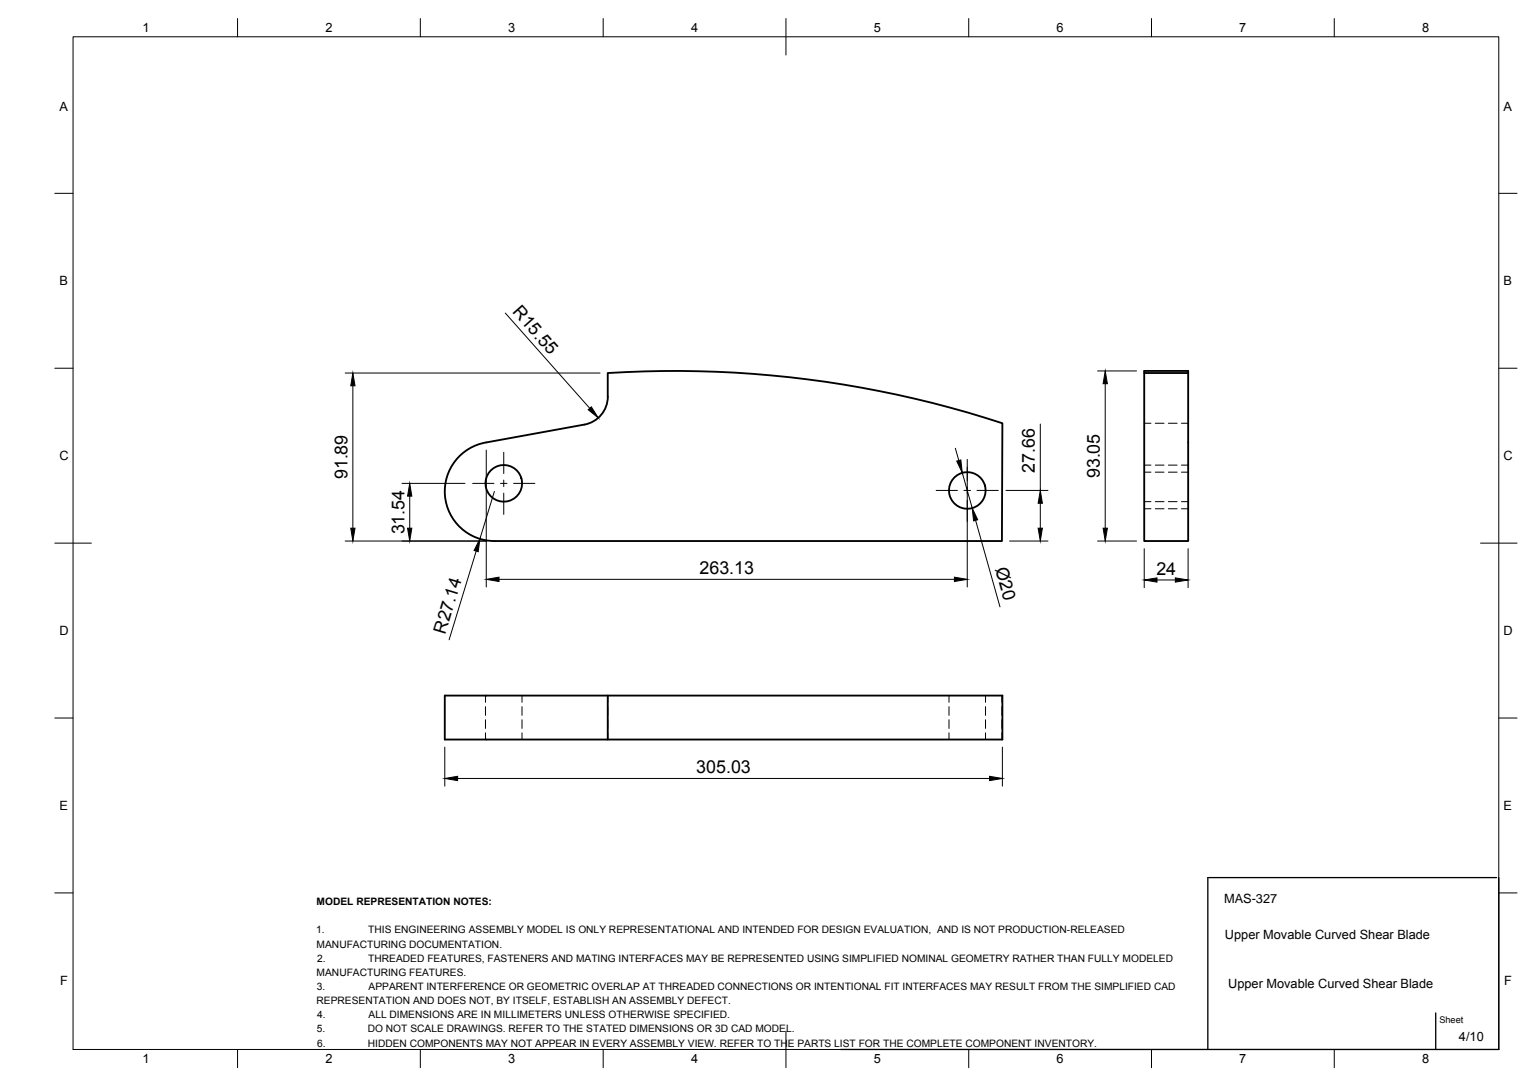
ISO-10303-21;
HEADER;
FILE_DESCRIPTION (('STEP AP214'),
    '1' );
FILE_NAME ('Upper Movable Curved Shear Blade.step',
    '2026-10-06T22:16:42',
    ( '' ),
    ( '' ),
    'SwSTEP 2.0',
    'SolidWorks 2025',
    '' );
FILE_SCHEMA (( 'AUTOMOTIVE_DESIGN' ));
ENDSEC;

DATA;
#48=FACE_BOUND ( 'NONE', #8175, .T. ) ;
#84=VECTOR ( 'NONE', #11009, 1000.000000000000000 ) ;
#209=CIRCLE ( 'NONE', #14661, 576.1986910693910886 ) ;
#225=ORIENTED_EDGE ( 'NONE', *, *, #21350, .F. ) ;
#238=EDGE_CURVE ( 'NONE', #951, #16393, #2471, .T. ) ;
#293=DIRECTION ( 'NONE',  ( -0.9609212714474144601, -0.2768218020313507610, 0.000000000000000000 ) ) ;
#337=ORIENTED_EDGE ( 'NONE', *, *, #13071, .F. ) ;
#354=DIRECTION ( 'NONE',  ( 0.000000000000000000, 0.000000000000000000, 1.000000000000000000 ) ) ;
#375=CLOSED_SHELL ( 'NONE', ( #8062, #8739, #16372, #2106, #6229, #2878, #10037, #18884, #18118, #3960, #13156, #6514, #20224, #19647 ) ) ;
#400=DIRECTION ( 'NONE',  ( 1.000000000000000000, 0.000000000000000000, 0.000000000000000000 ) ) ;
#488=VERTEX_POINT ( 'NONE', #17503 ) ;
#507=CARTESIAN_POINT ( 'NONE',  ( 180.1254907973641934, 54.87273858953557237, 4.000000000000021316 ) ) ;
#570=ORIENTED_EDGE ( 'NONE', *, *, #6351, .T. ) ;
#625=EDGE_LOOP ( 'NONE', ( #14044, #7065, #9180, #16970 ) ) ;
#792=EDGE_LOOP ( 'NONE', ( #7745, #13828, #225, #21173 ) ) ;
#896=ORIENTED_EDGE ( 'NONE', *, *, #16906, .F. ) ;
#935=DIRECTION ( 'NONE',  ( 1.000000000000000000, 0.000000000000000000, 0.000000000000000000 ) ) ;
#951=VERTEX_POINT ( 'NONE', #1744 ) ;
#964=CYLINDRICAL_SURFACE ( 'NONE', #11411, 10.00000000000000888 ) ;
#975=AXIS2_PLACEMENT_3D ( 'NONE', #5264, #5469, #6716 ) ;
#1029=FACE_OUTER_BOUND ( 'NONE', #6208, .T. ) ;
#1042=STYLED_ITEM ( 'NONE', ( #2053 ), #21529 ) ;
#1044=CARTESIAN_POINT ( 'NONE',  ( 161.4773229304660731, 84.89323405393692212, 4.000000000000021316 ) ) ;
#1179=DIRECTION ( 'NONE',  ( -0.000000000000000000, -0.000000000000000000, -1.000000000000000000 ) ) ;
#1205=FACE_OUTER_BOUND ( 'NONE', #8630, .T. ) ;
#1253=DIRECTION ( 'NONE',  ( -0.9599098561846887145, -0.2803088796301151375, 0.000000000000000000 ) ) ;
#1266=AXIS2_PLACEMENT_3D ( 'NONE', #2104, #12019, #2214 ) ;
#1272=EDGE_CURVE ( 'NONE', #951, #12140, #21577, .T. ) ;
#1305=VERTEX_POINT ( 'NONE', #9789 ) ;
#1307=FACE_OUTER_BOUND ( 'NONE', #18026, .T. ) ;
#1322=VECTOR ( 'NONE', #10602, 1000.000000000000000 ) ;
#1342=AXIS2_PLACEMENT_3D ( 'NONE', #8297, #20202, #15234 ) ;
#1409=APPLICATION_CONTEXT ( 'automotive_design' ) ;
#1477=CARTESIAN_POINT ( 'NONE',  ( 180.1254907973641934, 54.87273858953557237, 4.000000000000021316 ) ) ;
#1578=ORIENTED_EDGE ( 'NONE', *, *, #8963, .T. ) ;
#1633=CIRCLE ( 'NONE', #16042, 9.999999999999994671 ) ;
#1716=ORIENTED_EDGE ( 'NONE', *, *, #20163, .F. ) ;
#1717=EDGE_CURVE ( 'NONE', #16694, #21813, #4400, .T. ) ;
#1744=CARTESIAN_POINT ( 'NONE',  ( -104.7439762501682736, 39.86119447055682485, 4.000000000000021316 ) ) ;
#1816=UNCERTAINTY_MEASURE_WITH_UNIT (LENGTH_MEASURE( 1.000000000000000082E-05 ), #4027, 'distance_accuracy_value', 'NONE');
#1879=ORIENTED_EDGE ( 'NONE', *, *, #19571, .F. ) ;
#1905=VERTEX_POINT ( 'NONE', #7889 ) ;
#1914=EDGE_CURVE ( 'NONE', #10160, #15098, #7604, .T. ) ;
#1954=CARTESIAN_POINT ( 'NONE',  ( -94.10404323627655288, -13.18023274290474767, 4.000000000000021316 ) ) ;
#1980=CARTESIAN_POINT ( 'NONE',  ( 161.4773229304660731, 84.89323405393692212, -19.99999999999997868 ) ) ;
#2053=PRESENTATION_STYLE_ASSIGNMENT (( #7561 ) ) ;
#2104=CARTESIAN_POINT ( 'NONE',  ( -38.21168032741934439, -23.19216891395253910, -19.99999999999997868 ) ) ;
#2106=ADVANCED_FACE ( 'NONE', ( #48, #13498, #17116 ), #16685, .T. ) ;
#2150=ORIENTED_EDGE ( 'NONE', *, *, #9010, .T. ) ;
#2168=CARTESIAN_POINT ( 'NONE',  ( 180.1254907973641934, 54.87273858953557237, 4.000000000000021316 ) ) ;
#2187=VECTOR ( 'NONE', #12158, 1000.000000000000000 ) ;
#2214=DIRECTION ( 'NONE',  ( -1.000000000000000000, 0.000000000000000000, 0.000000000000000000 ) ) ;
#2361=VERTEX_POINT ( 'NONE', #6415 ) ;
#2403=CARTESIAN_POINT ( 'NONE',  ( 0.000000000000000000, 0.000000000000000000, 0.000000000000000000 ) ) ;
#2471=CIRCLE ( 'NONE', #12318, 27.14138364107347812 ) ;
#2487=CYLINDRICAL_SURFACE ( 'NONE', #17723, 10.00000000000000888 ) ;
#2538=CARTESIAN_POINT ( 'NONE',  ( 162.0641828542163125, 116.7231784796025948, -19.99999999999997868 ) ) ;
#2579=DIRECTION ( 'NONE',  ( 0.2768218020313508165, -0.9609212714474144601, 0.000000000000000000 ) ) ;
#2664=EDGE_CURVE ( 'NONE', #10827, #15137, #5819, .T. ) ;
#2733=DIRECTION ( 'NONE',  ( 0.9949940778855791423, 0.09993390301907582873, 0.000000000000000000 ) ) ;
#2843=LINE ( 'NONE', #18047, #84 ) ;
#2876=CIRCLE ( 'NONE', #14842, 9.999999999999994671 ) ;
#2878=ADVANCED_FACE ( 'NONE', ( #1205 ), #16736, .T. ) ;
#3049=DIRECTION ( 'NONE',  ( 1.000000000000000000, 0.000000000000000000, -0.000000000000000000 ) ) ;
#3238=AXIS2_PLACEMENT_3D ( 'NONE', #19808, #9892, #3049 ) ;
#3242=CARTESIAN_POINT ( 'NONE',  ( -101.1064508287285832, 10.96617311717548660, 4.000000000000021316 ) ) ;
#3459=EDGE_LOOP ( 'NONE', ( #7718, #4157, #7317, #15466 ) ) ;
#3466=EDGE_CURVE ( 'NONE', #9506, #10827, #4066, .T. ) ;
#3570=VERTEX_POINT ( 'NONE', #12547 ) ;
#3591=EDGE_CURVE ( 'NONE', #4466, #7553, #14300, .T. ) ;
#3672=ORIENTED_EDGE ( 'NONE', *, *, #238, .T. ) ;
#3713=AXIS2_PLACEMENT_3D ( 'NONE', #9112, #4032, #935 ) ;
#3776=EDGE_LOOP ( 'NONE', ( #15667, #19204 ) ) ;
#3783=ORIENTED_EDGE ( 'NONE', *, *, #14965, .F. ) ;
#3812=ORIENTED_EDGE ( 'NONE', *, *, #238, .F. ) ;
#3867=( GEOMETRIC_REPRESENTATION_CONTEXT ( 3 ) GLOBAL_UNCERTAINTY_ASSIGNED_CONTEXT ( ( #1816 ) ) GLOBAL_UNIT_ASSIGNED_CONTEXT ( ( #4027, #8894, #9109 ) ) REPRESENTATION_CONTEXT ( 'NONE', 'WORKASPACE' ) );
#3877=LINE ( 'NONE', #5737, #1322 ) ;
#3886=PRODUCT_DEFINITION_FORMATION_WITH_SPECIFIED_SOURCE ( 'ANY', '', #9956, .NOT_KNOWN. ) ;
#3924=CARTESIAN_POINT ( 'NONE',  ( 151.4773229304660731, 84.89323405393692212, -19.99999999999997868 ) ) ;
#3942=ORIENTED_EDGE ( 'NONE', *, *, #8167, .F. ) ;
#3960=ADVANCED_FACE ( 'NONE', ( #13848 ), #20583, .T. ) ;
#4027=( LENGTH_UNIT ( ) NAMED_UNIT ( * ) SI_UNIT ( .MILLI., .METRE. ) );
#4029=EDGE_CURVE ( 'NONE', #20969, #10160, #18710, .T. ) ;
#4032=DIRECTION ( 'NONE',  ( 0.000000000000000000, 0.000000000000000000, 1.000000000000000000 ) ) ;
#4041=FACE_OUTER_BOUND ( 'NONE', #14824, .T. ) ;
#4059=DIRECTION ( 'NONE',  ( -0.9949940778855791423, -0.09993390301907582873, 0.000000000000000000 ) ) ;
#4066=LINE ( 'NONE', #21045, #18173 ) ;
#4099=AXIS2_PLACEMENT_3D ( 'NONE', #10030, #8156, #14861 ) ;
#4128=ORIENTED_EDGE ( 'NONE', *, *, #10231, .T. ) ;
#4157=ORIENTED_EDGE ( 'NONE', *, *, #6919, .F. ) ;
#4183=VERTEX_POINT ( 'NONE', #2168 ) ;
#4196=CARTESIAN_POINT ( 'NONE',  ( 151.4773229304660731, 84.89323405393692212, 4.000000000000021316 ) ) ;
#4226=CYLINDRICAL_SURFACE ( 'NONE', #7967, 9.999999999999994671 ) ;
#4231=EDGE_CURVE ( 'NONE', #10160, #10827, #7575, .T. ) ;
#4258=EDGE_CURVE ( 'NONE', #15220, #21430, #19462, .T. ) ;
#4284=PRODUCT_DEFINITION_SHAPE ( 'NONE', 'NONE',  #20915 ) ;
#4327=DIRECTION ( 'NONE',  ( -0.000000000000000000, -0.000000000000000000, -1.000000000000000000 ) ) ;
#4350=CARTESIAN_POINT ( 'NONE',  ( 180.1254907973641934, 54.87273858953557237, -19.99999999999997868 ) ) ;
#4383=ORIENTED_EDGE ( 'NONE', *, *, #6351, .F. ) ;
#4400=CIRCLE ( 'NONE', #3713, 9.999999999999994671 ) ;
#4403=ORIENTED_EDGE ( 'NONE', *, *, #8525, .T. ) ;
#4466=VERTEX_POINT ( 'NONE', #11295 ) ;
#4508=DIRECTION ( 'NONE',  ( -1.000000000000000000, 0.000000000000000000, 0.000000000000000000 ) ) ;
#4562=DIRECTION ( 'NONE',  ( -0.000000000000000000, -0.000000000000000000, -1.000000000000000000 ) ) ;
#4585=FACE_BOUND ( 'NONE', #17508, .T. ) ;
#4591=DIRECTION ( 'NONE',  ( -1.000000000000000000, 0.000000000000000000, 0.000000000000000000 ) ) ;
#4638=AXIS2_PLACEMENT_3D ( 'NONE', #18358, #13178, #19910 ) ;
#4642=DIRECTION ( 'NONE',  ( 1.000000000000000000, 0.000000000000000000, 0.000000000000000000 ) ) ;
#4701=DIRECTION ( 'NONE',  ( -0.000000000000000000, -0.000000000000000000, -1.000000000000000000 ) ) ;
#4739=DIRECTION ( 'NONE',  ( 1.000000000000000000, 0.000000000000000000, 0.000000000000000000 ) ) ;
#4768=DIRECTION ( 'NONE',  ( 0.000000000000000000, 0.000000000000000000, 1.000000000000000000 ) ) ;
#4782=DIRECTION ( 'NONE',  ( 0.000000000000000000, 0.000000000000000000, 1.000000000000000000 ) ) ;
#4806=DIRECTION ( 'NONE',  ( 1.000000000000000000, 0.000000000000000000, 0.000000000000000000 ) ) ;
#4831=CYLINDRICAL_SURFACE ( 'NONE', #9491, 9.999999999999994671 ) ;
#4872=LINE ( 'NONE', #16542, #5060 ) ;
#5060=VECTOR ( 'NONE', #21745, 1000.000000000000000 ) ;
#5264=CARTESIAN_POINT ( 'NONE',  ( -143.7724355939531904, 531.4176628826018032, 4.000000000000021316 ) ) ;
#5334=CARTESIAN_POINT ( 'NONE',  ( -97.23064952102208736, 13.78046159333444720, 4.000000000000021316 ) ) ;
#5357=CARTESIAN_POINT ( 'NONE',  ( -19.70755683829218796, -31.26594044116892590, -19.99999999999997868 ) ) ;
#5385=CARTESIAN_POINT ( 'NONE',  ( -81.10645082872859746, 10.96617311717548837, -19.99999999999997868 ) ) ;
#5436=CARTESIAN_POINT ( 'NONE',  ( -23.27144139456156324, -18.88988604584387332, -19.99999999999997868 ) ) ;
#5462=VECTOR ( 'NONE', #1179, 1000.000000000000000 ) ;
#5469=DIRECTION ( 'NONE',  ( -0.000000000000000000, -0.000000000000000000, -1.000000000000000000 ) ) ;
#5555=EDGE_CURVE ( 'NONE', #13376, #488, #6969, .T. ) ;
#5607=EDGE_CURVE ( 'NONE', #1905, #21813, #3877, .T. ) ;
#5629=VERTEX_POINT ( 'NONE', #2538 ) ;
#5697=ORIENTED_EDGE ( 'NONE', *, *, #11604, .T. ) ;
#5737=CARTESIAN_POINT ( 'NONE',  ( -81.10645082872859746, 10.96617311717548837, 4.000000000000021316 ) ) ;
#5819=CIRCLE ( 'NONE', #1266, 15.54735917280169311 ) ;
#6027=CARTESIAN_POINT ( 'NONE',  ( -94.10404323627655288, -13.18023274290474767, 4.000000000000021316 ) ) ;
#6077=CARTESIAN_POINT ( 'NONE',  ( -91.10645082872859746, 10.96617311717548660, 4.000000000000021316 ) ) ;
#6114=CARTESIAN_POINT ( 'NONE',  ( -97.23064952102208736, 13.78046159333444720, 4.000000000000021316 ) ) ;
#6149=DIRECTION ( 'NONE',  ( -0.000000000000000000, -0.000000000000000000, -1.000000000000000000 ) ) ;
#6194=ORIENTED_EDGE ( 'NONE', *, *, #2664, .T. ) ;
#6208=EDGE_LOOP ( 'NONE', ( #11910, #13559, #15642, #3783 ) ) ;
#6229=ADVANCED_FACE ( 'NONE', ( #16482, #4585, #11305 ), #6355, .F. ) ;
#6239=AXIS2_PLACEMENT_3D ( 'NONE', #4196, #354, #18974 ) ;
#6351=EDGE_CURVE ( 'NONE', #21430, #2361, #11676, .T. ) ;
#6355=PLANE ( 'NONE',  #3238 ) ;
#6409=AXIS2_PLACEMENT_3D ( 'NONE', #13412, #20146, #400 ) ;
#6415=CARTESIAN_POINT ( 'NONE',  ( 180.1254907973641934, 54.87273858953557237, -19.99999999999997868 ) ) ;
#6446=SHAPE_DEFINITION_REPRESENTATION ( #4284, #15921 ) ;
#6455=CYLINDRICAL_SURFACE ( 'NONE', #4638, 27.14138364107347812 ) ;
#6505=VECTOR ( 'NONE', #11206, 1000.000000000000000 ) ;
#6514=ADVANCED_FACE ( 'NONE', ( #17353 ), #20891, .F. ) ;
#6609=EDGE_CURVE ( 'NONE', #12140, #1305, #21556, .T. ) ;
#6661=EDGE_CURVE ( 'NONE', #13376, #7553, #16350, .T. ) ;
#6704=LINE ( 'NONE', #13411, #12909 ) ;
#6716=DIRECTION ( 'NONE',  ( -1.000000000000000000, 0.000000000000000000, 0.000000000000000000 ) ) ;
#6919=EDGE_CURVE ( 'NONE', #3570, #5629, #11722, .T. ) ;
#6969=CIRCLE ( 'NONE', #6239, 10.00000000000000888 ) ;
#7037=( GEOMETRIC_REPRESENTATION_CONTEXT ( 3 ) GLOBAL_UNCERTAINTY_ASSIGNED_CONTEXT ( ( #8652 ) ) GLOBAL_UNIT_ASSIGNED_CONTEXT ( ( #20926, #7378, #12539 ) ) REPRESENTATION_CONTEXT ( 'NONE', 'WORKASPACE' ) );
#7050=DIRECTION ( 'NONE',  ( 0.000000000000000000, 0.000000000000000000, 1.000000000000000000 ) ) ;
#7065=ORIENTED_EDGE ( 'NONE', *, *, #4231, .F. ) ;
#7107=CARTESIAN_POINT ( 'NONE',  ( -104.7439762501682736, 39.86119447055682485, -19.99999999999997868 ) ) ;
#7258=ORIENTED_EDGE ( 'NONE', *, *, #4029, .T. ) ;
#7317=ORIENTED_EDGE ( 'NONE', *, *, #10231, .F. ) ;
#7378=( NAMED_UNIT ( * ) PLANE_ANGLE_UNIT ( ) SI_UNIT ( $, .RADIAN. ) );
#7419=ORIENTED_EDGE ( 'NONE', *, *, #6661, .F. ) ;
#7451=CARTESIAN_POINT ( 'NONE',  ( -97.23064952102208736, 13.78046159333444720, -19.99999999999997868 ) ) ;
#7471=VECTOR ( 'NONE', #19881, 1000.000000000000000 ) ;
#7501=ORIENTED_EDGE ( 'NONE', *, *, #4258, .T. ) ;
#7553=VERTEX_POINT ( 'NONE', #1980 ) ;
#7561=SURFACE_STYLE_USAGE ( .BOTH. , #17460 ) ;
#7575=LINE ( 'NONE', #14275, #12948 ) ;
#7582=ORIENTED_EDGE ( 'NONE', *, *, #20163, .T. ) ;
#7604=CIRCLE ( 'NONE', #9361, 15.54735917280169311 ) ;
#7638=AXIS2_PLACEMENT_3D ( 'NONE', #19275, #10905, #17608 ) ;
#7678=VECTOR ( 'NONE', #15407, 1000.000000000000114 ) ;
#7718=ORIENTED_EDGE ( 'NONE', *, *, #8167, .T. ) ;
#7745=ORIENTED_EDGE ( 'NONE', *, *, #16946, .T. ) ;
#7789=DIRECTION ( 'NONE',  ( 0.000000000000000000, 0.000000000000000000, 1.000000000000000000 ) ) ;
#7809=PLANE ( 'NONE',  #17114 ) ;
#7889=CARTESIAN_POINT ( 'NONE',  ( -81.10645082872859746, 10.96617311717548837, 4.000000000000021316 ) ) ;
#7954=DIRECTION ( 'NONE',  ( 0.000000000000000000, 0.000000000000000000, 1.000000000000000000 ) ) ;
#7961=AXIS2_PLACEMENT_3D ( 'NONE', #5334, #20552, #20229 ) ;
#7967=AXIS2_PLACEMENT_3D ( 'NONE', #8982, #4327, #11052 ) ;
#8018=CARTESIAN_POINT ( 'NONE',  ( -94.10404323627655288, -13.18023274290474767, 4.000000000000021316 ) ) ;
#8062=ADVANCED_FACE ( 'NONE', ( #4041 ), #2487, .F. ) ;
#8121=EDGE_LOOP ( 'NONE', ( #10128, #20673, #1578, #1879 ) ) ;
#8131=EDGE_CURVE ( 'NONE', #16393, #20969, #19854, .T. ) ;
#8156=DIRECTION ( 'NONE',  ( -0.000000000000000000, -0.000000000000000000, -1.000000000000000000 ) ) ;
#8167=EDGE_CURVE ( 'NONE', #2361, #5629, #17793, .T. ) ;
#8175=EDGE_LOOP ( 'NONE', ( #14150, #17505 ) ) ;
#8195=ORIENTED_EDGE ( 'NONE', *, *, #1914, .F. ) ;
#8297=CARTESIAN_POINT ( 'NONE',  ( -97.23064952102208736, 13.78046159333444720, -19.99999999999997868 ) ) ;
#8335=CARTESIAN_POINT ( 'NONE',  ( -124.3720331620955619, 13.78046159333444720, 4.000000000000021316 ) ) ;
#8525=EDGE_CURVE ( 'NONE', #488, #4466, #12273, .T. ) ;
#8630=EDGE_LOOP ( 'NONE', ( #19998, #3812, #10096, #19794 ) ) ;
#8652=UNCERTAINTY_MEASURE_WITH_UNIT (LENGTH_MEASURE( 1.000000000000000082E-05 ), #20926, 'distance_accuracy_value', 'NONE');
#8739=ADVANCED_FACE ( 'NONE', ( #1029 ), #4226, .F. ) ;
#8833=ORIENTED_EDGE ( 'NONE', *, *, #2664, .F. ) ;
#8894=( NAMED_UNIT ( * ) PLANE_ANGLE_UNIT ( ) SI_UNIT ( $, .RADIAN. ) );
#8963=EDGE_CURVE ( 'NONE', #1305, #9506, #17520, .T. ) ;
#8982=CARTESIAN_POINT ( 'NONE',  ( -91.10645082872859746, 10.96617311717548660, 4.000000000000021316 ) ) ;
#9010=EDGE_CURVE ( 'NONE', #15098, #15137, #4872, .T. ) ;
#9038=AXIS2_PLACEMENT_3D ( 'NONE', #1477, #1253, #18227 ) ;
#9086=EDGE_CURVE ( 'NONE', #15220, #4183, #209, .T. ) ;
#9109=( NAMED_UNIT ( * ) SI_UNIT ( $, .STERADIAN. ) SOLID_ANGLE_UNIT ( ) );
#9112=CARTESIAN_POINT ( 'NONE',  ( -91.10645082872859746, 10.96617311717548660, -19.99999999999997868 ) ) ;
#9180=ORIENTED_EDGE ( 'NONE', *, *, #4029, .F. ) ;
#9238=ORIENTED_EDGE ( 'NONE', *, *, #6609, .F. ) ;
#9240=AXIS2_PLACEMENT_3D ( 'NONE', #15914, #2579, #18911 ) ;
#9361=AXIS2_PLACEMENT_3D ( 'NONE', #21226, #9544, #13166 ) ;
#9364=ORIENTED_EDGE ( 'NONE', *, *, #3466, .F. ) ;
#9491=AXIS2_PLACEMENT_3D ( 'NONE', #21270, #6149, #19604 ) ;
#9506=VERTEX_POINT ( 'NONE', #17628 ) ;
#9509=VECTOR ( 'NONE', #293, 1000.000000000000000 ) ;
#9544=DIRECTION ( 'NONE',  ( -0.000000000000000000, -0.000000000000000000, -1.000000000000000000 ) ) ;
#9789=CARTESIAN_POINT ( 'NONE',  ( -124.3720331620955619, 13.78046159333444720, -19.99999999999997868 ) ) ;
#9866=PLANE ( 'NONE',  #18383 ) ;
#9892=DIRECTION ( 'NONE',  ( 0.000000000000000000, 0.000000000000000000, 1.000000000000000000 ) ) ;
#9933=ORIENTED_EDGE ( 'NONE', *, *, #19774, .F. ) ;
#9953=DIRECTION ( 'NONE',  ( 1.000000000000000000, 0.000000000000000000, 0.000000000000000000 ) ) ;
#9956=PRODUCT ( 'Upper Movable Curved Shear Blade', 'Upper Movable Curved Shear Blade', '', ( #16687 ) ) ;
#9978=DIRECTION ( 'NONE',  ( -0.2767211344570352782, 0.9609502660100632809, 0.000000000000000000 ) ) ;
#10030=CARTESIAN_POINT ( 'NONE',  ( -97.23064952102208736, 13.78046159333444720, 4.000000000000021316 ) ) ;
#10037=ADVANCED_FACE ( 'NONE', ( #19159 ), #7809, .F. ) ;
#10039=VECTOR ( 'NONE', #15289, 1000.000000000000000 ) ;
#10096=ORIENTED_EDGE ( 'NONE', *, *, #1272, .T. ) ;
#10128=ORIENTED_EDGE ( 'NONE', *, *, #8131, .F. ) ;
#10160=VERTEX_POINT ( 'NONE', #16923 ) ;
#10202=CARTESIAN_POINT ( 'NONE',  ( -19.70755683829218796, -31.26594044116892590, 4.000000000000021316 ) ) ;
#10203=AXIS2_PLACEMENT_3D ( 'NONE', #15167, #15394, #4806 ) ;
#10209=EDGE_LOOP ( 'NONE', ( #7419, #20028, #4403, #20431 ) ) ;
#10231=EDGE_CURVE ( 'NONE', #4183, #3570, #6704, .T. ) ;
#10303=CARTESIAN_POINT ( 'NONE',  ( 162.0641828542163125, 116.7231784796025948, 4.000000000000021316 ) ) ;
#10328=DIRECTION ( 'NONE',  ( -0.2803088796301151375, 0.9599098561846886035, 0.000000000000000000 ) ) ;
#10357=SHAPE_REPRESENTATION_RELATIONSHIP ( 'NONE' , 'NONE' ,  #15921, #12417 ) ;
#10389=PRODUCT_DEFINITION_CONTEXT ( 'detailed design', #13918, 'design' ) ;
#10530=CARTESIAN_POINT ( 'NONE',  ( 141.4773229304660447, 84.89323405393692212, 4.000000000000021316 ) ) ;
#10602=DIRECTION ( 'NONE',  ( -0.000000000000000000, -0.000000000000000000, -1.000000000000000000 ) ) ;
#10827=VERTEX_POINT ( 'NONE', #13888 ) ;
#10905=DIRECTION ( 'NONE',  ( 0.000000000000000000, 0.000000000000000000, 1.000000000000000000 ) ) ;
#11009=DIRECTION ( 'NONE',  ( -0.000000000000000000, -0.000000000000000000, -1.000000000000000000 ) ) ;
#11052=DIRECTION ( 'NONE',  ( -1.000000000000000000, 0.000000000000000000, 0.000000000000000000 ) ) ;
#11127=DIRECTION ( 'NONE',  ( -0.000000000000000000, -0.000000000000000000, -1.000000000000000000 ) ) ;
#11129=CIRCLE ( 'NONE', #20301, 9.999999999999994671 ) ;
#11147=DIRECTION ( 'NONE',  ( 0.000000000000000000, 0.000000000000000000, 1.000000000000000000 ) ) ;
#11206=DIRECTION ( 'NONE',  ( -0.000000000000000000, -0.000000000000000000, -1.000000000000000000 ) ) ;
#11295=CARTESIAN_POINT ( 'NONE',  ( 141.4773229304660447, 84.89323405393692212, -19.99999999999997868 ) ) ;
#11305=FACE_BOUND ( 'NONE', #11791, .T. ) ;
#11338=VECTOR ( 'NONE', #13594, 1000.000000000000000 ) ;
#11387=LINE ( 'NONE', #19546, #17461 ) ;
#11403=CARTESIAN_POINT ( 'NONE',  ( -19.70755683829218796, -31.26594044116892590, 4.000000000000021316 ) ) ;
#11411=AXIS2_PLACEMENT_3D ( 'NONE', #12976, #4701, #4591 ) ;
#11604=EDGE_CURVE ( 'NONE', #7553, #4466, #14333, .T. ) ;
#11618=CARTESIAN_POINT ( 'NONE',  ( -23.27144139456156324, -18.88988604584387332, 4.000000000000021316 ) ) ;
#11676=CIRCLE ( 'NONE', #6409, 576.1986910693910886 ) ;
#11722=LINE ( 'NONE', #10303, #11338 ) ;
#11729=CARTESIAN_POINT ( 'NONE',  ( -124.3720331620955619, 13.78046159333444720, 4.000000000000021316 ) ) ;
#11791=EDGE_LOOP ( 'NONE', ( #16443, #5697 ) ) ;
#11910=ORIENTED_EDGE ( 'NONE', *, *, #13655, .T. ) ;
#11971=CARTESIAN_POINT ( 'NONE',  ( 162.0641828542163125, 116.7231784796025948, 4.000000000000021316 ) ) ;
#12019=DIRECTION ( 'NONE',  ( -0.000000000000000000, -0.000000000000000000, -1.000000000000000000 ) ) ;
#12041=AXIS2_PLACEMENT_3D ( 'NONE', #7451, #4782, #12832 ) ;
#12140=VERTEX_POINT ( 'NONE', #7107 ) ;
#12144=CARTESIAN_POINT ( 'NONE',  ( -23.27144139456156324, -18.88988604584387332, -19.99999999999997868 ) ) ;
#12158=DIRECTION ( 'NONE',  ( -0.000000000000000000, -0.000000000000000000, -1.000000000000000000 ) ) ;
#12177=FILL_AREA_STYLE ('',( #19024 ) ) ;
#12273=LINE ( 'NONE', #10530, #20984 ) ;
#12303=MECHANICAL_DESIGN_GEOMETRIC_PRESENTATION_REPRESENTATION('',(#1042),#3867);
#12318=AXIS2_PLACEMENT_3D ( 'NONE', #16310, #7954, #4739 ) ;
#12365=DIRECTION ( 'NONE',  ( 0.000000000000000000, 0.000000000000000000, 1.000000000000000000 ) ) ;
#12417=ADVANCED_BREP_SHAPE_REPRESENTATION ( '', ( #21529, #12657 ), #7037 ) ;
#12498=CARTESIAN_POINT ( 'NONE',  ( -101.1064508287285832, 10.96617311717548660, -19.99999999999997868 ) ) ;
#12510=SURFACE_STYLE_FILL_AREA ( #12177 ) ;
#12522=CARTESIAN_POINT ( 'NONE',  ( 151.4773229304660731, 84.89323405393692212, 4.000000000000021316 ) ) ;
#12539=( NAMED_UNIT ( * ) SI_UNIT ( $, .STERADIAN. ) SOLID_ANGLE_UNIT ( ) );
#12541=DIRECTION ( 'NONE',  ( -0.09993390301907582873, 0.9949940778855791423, 0.000000000000000000 ) ) ;
#12547=CARTESIAN_POINT ( 'NONE',  ( 162.0641828542163125, 116.7231784796025948, 4.000000000000021316 ) ) ;
#12576=AXIS2_PLACEMENT_3D ( 'NONE', #3924, #20358, #20681 ) ;
#12649=FACE_OUTER_BOUND ( 'NONE', #10209, .T. ) ;
#12657=AXIS2_PLACEMENT_3D ( 'NONE', #2403, #7050, #17169 ) ;
#12832=DIRECTION ( 'NONE',  ( 1.000000000000000000, 0.000000000000000000, 0.000000000000000000 ) ) ;
#12909=VECTOR ( 'NONE', #10328, 1000.000000000000114 ) ;
#12948=VECTOR ( 'NONE', #17367, 1000.000000000000000 ) ;
#12976=CARTESIAN_POINT ( 'NONE',  ( 151.4773229304660731, 84.89323405393692212, 4.000000000000021316 ) ) ;
#13071=EDGE_CURVE ( 'NONE', #15098, #15220, #11387, .T. ) ;
#13131=ORIENTED_EDGE ( 'NONE', *, *, #1914, .T. ) ;
#13156=ADVANCED_FACE ( 'NONE', ( #16346 ), #20009, .F. ) ;
#13166=DIRECTION ( 'NONE',  ( -1.000000000000000000, 0.000000000000000000, 0.000000000000000000 ) ) ;
#13176=ORIENTED_EDGE ( 'NONE', *, *, #8525, .F. ) ;
#13178=DIRECTION ( 'NONE',  ( -0.000000000000000000, -0.000000000000000000, -1.000000000000000000 ) ) ;
#13229=VERTEX_POINT ( 'NONE', #3242 ) ;
#13265=LINE ( 'NONE', #15018, #7471 ) ;
#13280=FACE_OUTER_BOUND ( 'NONE', #21297, .T. ) ;
#13301=VECTOR ( 'NONE', #21677, 1000.000000000000000 ) ;
#13376=VERTEX_POINT ( 'NONE', #15139 ) ;
#13411=CARTESIAN_POINT ( 'NONE',  ( 180.1254907973641934, 54.87273858953557237, 4.000000000000021316 ) ) ;
#13412=CARTESIAN_POINT ( 'NONE',  ( -143.7724355939531904, 531.4176628826018032, -19.99999999999997868 ) ) ;
#13498=FACE_OUTER_BOUND ( 'NONE', #13788, .T. ) ;
#13559=ORIENTED_EDGE ( 'NONE', *, *, #5607, .T. ) ;
#13594=DIRECTION ( 'NONE',  ( -0.000000000000000000, -0.000000000000000000, -1.000000000000000000 ) ) ;
#13655=EDGE_CURVE ( 'NONE', #13229, #1905, #11129, .T. ) ;
#13694=ORIENTED_EDGE ( 'NONE', *, *, #5607, .F. ) ;
#13788=EDGE_LOOP ( 'NONE', ( #3672, #17546, #7258, #13131, #21125, #13879, #4128, #15935 ) ) ;
#13803=LINE ( 'NONE', #12144, #20056 ) ;
#13828=ORIENTED_EDGE ( 'NONE', *, *, #1272, .F. ) ;
#13847=EDGE_CURVE ( 'NONE', #1905, #13229, #1633, .T. ) ;
#13848=FACE_OUTER_BOUND ( 'NONE', #21516, .T. ) ;
#13879=ORIENTED_EDGE ( 'NONE', *, *, #9086, .T. ) ;
#13888=CARTESIAN_POINT ( 'NONE',  ( -39.76538861119684753, -7.722638610254815461, -19.99999999999997868 ) ) ;
#13918=APPLICATION_CONTEXT ( 'automotive_design' ) ;
#14044=ORIENTED_EDGE ( 'NONE', *, *, #3466, .T. ) ;
#14062=DIRECTION ( 'NONE',  ( -0.2803088796301151375, 0.9599098561846886035, 0.000000000000000000 ) ) ;
#14150=ORIENTED_EDGE ( 'NONE', *, *, #13655, .F. ) ;
#14202=ORIENTED_EDGE ( 'NONE', *, *, #16946, .F. ) ;
#14275=CARTESIAN_POINT ( 'NONE',  ( -39.76538861119684753, -7.722638610254815461, 4.000000000000021316 ) ) ;
#14300=CIRCLE ( 'NONE', #7638, 10.00000000000000888 ) ;
#14333=CIRCLE ( 'NONE', #12576, 10.00000000000000888 ) ;
#14515=CARTESIAN_POINT ( 'NONE',  ( -94.10404323627655288, -13.18023274290474767, 4.000000000000021316 ) ) ;
#14646=CYLINDRICAL_SURFACE ( 'NONE', #19168, 15.54735917280169311 ) ;
#14661=AXIS2_PLACEMENT_3D ( 'NONE', #18203, #15118, #9953 ) ;
#14820=FACE_OUTER_BOUND ( 'NONE', #8121, .T. ) ;
#14824=EDGE_LOOP ( 'NONE', ( #17348, #15438, #17640, #13176 ) ) ;
#14842=AXIS2_PLACEMENT_3D ( 'NONE', #21538, #4768, #16446 ) ;
#14861=DIRECTION ( 'NONE',  ( -1.000000000000000000, 0.000000000000000000, 0.000000000000000000 ) ) ;
#14965=EDGE_CURVE ( 'NONE', #13229, #16694, #2843, .T. ) ;
#15008=ORIENTED_EDGE ( 'NONE', *, *, #8963, .F. ) ;
#15018=CARTESIAN_POINT ( 'NONE',  ( 162.0641828542163125, 116.7231784796025948, -19.99999999999997868 ) ) ;
#15098=VERTEX_POINT ( 'NONE', #21267 ) ;
#15118=DIRECTION ( 'NONE',  ( 0.000000000000000000, 0.000000000000000000, 1.000000000000000000 ) ) ;
#15137=VERTEX_POINT ( 'NONE', #5436 ) ;
#15139=CARTESIAN_POINT ( 'NONE',  ( 161.4773229304660731, 84.89323405393692212, 4.000000000000021316 ) ) ;
#15163=EDGE_CURVE ( 'NONE', #16393, #1305, #17222, .T. ) ;
#15167=CARTESIAN_POINT ( 'NONE',  ( 151.4773229304660731, 84.89323405393692212, 4.000000000000021316 ) ) ;
#15220=VERTEX_POINT ( 'NONE', #10202 ) ;
#15234=DIRECTION ( 'NONE',  ( 1.000000000000000000, 0.000000000000000000, 0.000000000000000000 ) ) ;
#15289=DIRECTION ( 'NONE',  ( -0.000000000000000000, -0.000000000000000000, -1.000000000000000000 ) ) ;
#15394=DIRECTION ( 'NONE',  ( 0.000000000000000000, 0.000000000000000000, 1.000000000000000000 ) ) ;
#15407=DIRECTION ( 'NONE',  ( 0.9949940778855791423, 0.09993390301907582873, 0.000000000000000000 ) ) ;
#15438=ORIENTED_EDGE ( 'NONE', *, *, #6661, .T. ) ;
#15466=ORIENTED_EDGE ( 'NONE', *, *, #19774, .T. ) ;
#15642=ORIENTED_EDGE ( 'NONE', *, *, #1717, .F. ) ;
#15667=ORIENTED_EDGE ( 'NONE', *, *, #21147, .F. ) ;
#15914=CARTESIAN_POINT ( 'NONE',  ( 162.0641828542163125, 116.7231784796025948, 4.000000000000021316 ) ) ;
#15921=SHAPE_REPRESENTATION ( 'Upper Movable Curved Shear Blade', ( #12657 ), #7037 ) ;
#15935=ORIENTED_EDGE ( 'NONE', *, *, #21350, .T. ) ;
#16042=AXIS2_PLACEMENT_3D ( 'NONE', #6077, #11147, #4642 ) ;
#16147=DIRECTION ( 'NONE',  ( -0.000000000000000000, -0.000000000000000000, -1.000000000000000000 ) ) ;
#16190=CARTESIAN_POINT ( 'NONE',  ( -38.21168032741934439, -23.19216891395253910, 4.000000000000021316 ) ) ;
#16310=CARTESIAN_POINT ( 'NONE',  ( -97.23064952102208736, 13.78046159333444720, 4.000000000000021316 ) ) ;
#16346=FACE_OUTER_BOUND ( 'NONE', #3459, .T. ) ;
#16350=LINE ( 'NONE', #1044, #18388 ) ;
#16362=ORIENTED_EDGE ( 'NONE', *, *, #4258, .F. ) ;
#16372=ADVANCED_FACE ( 'NONE', ( #14820 ), #6455, .T. ) ;
#16393=VERTEX_POINT ( 'NONE', #8335 ) ;
#16443=ORIENTED_EDGE ( 'NONE', *, *, #3591, .T. ) ;
#16446=DIRECTION ( 'NONE',  ( 1.000000000000000000, 0.000000000000000000, 0.000000000000000000 ) ) ;
#16482=FACE_OUTER_BOUND ( 'NONE', #19308, .T. ) ;
#16507=LINE ( 'NONE', #11971, #9509 ) ;
#16542=CARTESIAN_POINT ( 'NONE',  ( -23.27144139456156324, -18.88988604584387332, 4.000000000000021316 ) ) ;
#16685=PLANE ( 'NONE',  #7961 ) ;
#16687=PRODUCT_CONTEXT ( 'NONE', #1409, 'mechanical' ) ;
#16694=VERTEX_POINT ( 'NONE', #12498 ) ;
#16736=CYLINDRICAL_SURFACE ( 'NONE', #4099, 27.14138364107347812 ) ;
#16906=EDGE_CURVE ( 'NONE', #21813, #16694, #2876, .T. ) ;
#16923=CARTESIAN_POINT ( 'NONE',  ( -39.76538861119684753, -7.722638610254815461, 4.000000000000021316 ) ) ;
#16946=EDGE_CURVE ( 'NONE', #5629, #12140, #13265, .T. ) ;
#16970=ORIENTED_EDGE ( 'NONE', *, *, #19571, .T. ) ;
#17074=ORIENTED_EDGE ( 'NONE', *, *, #9086, .F. ) ;
#17114=AXIS2_PLACEMENT_3D ( 'NONE', #14515, #12541, #4059 ) ;
#17116=FACE_BOUND ( 'NONE', #3776, .T. ) ;
#17169=DIRECTION ( 'NONE',  ( 1.000000000000000000, 0.000000000000000000, 0.000000000000000000 ) ) ;
#17222=LINE ( 'NONE', #11729, #2187 ) ;
#17228=DIRECTION ( 'NONE',  ( -0.000000000000000000, -0.000000000000000000, -1.000000000000000000 ) ) ;
#17234=ORIENTED_EDGE ( 'NONE', *, *, #16906, .T. ) ;
#17249=LINE ( 'NONE', #507, #10039 ) ;
#17348=ORIENTED_EDGE ( 'NONE', *, *, #21147, .T. ) ;
#17353=FACE_OUTER_BOUND ( 'NONE', #792, .T. ) ;
#17367=DIRECTION ( 'NONE',  ( -0.000000000000000000, -0.000000000000000000, -1.000000000000000000 ) ) ;
#17460=SURFACE_SIDE_STYLE ('',( #12510 ) ) ;
#17461=VECTOR ( 'NONE', #21544, 999.9999999999998863 ) ;
#17474=DIRECTION ( 'NONE',  ( 1.000000000000000000, 0.000000000000000000, 0.000000000000000000 ) ) ;
#17503=CARTESIAN_POINT ( 'NONE',  ( 141.4773229304660447, 84.89323405393692212, 4.000000000000021316 ) ) ;
#17505=ORIENTED_EDGE ( 'NONE', *, *, #13847, .F. ) ;
#17508=EDGE_LOOP ( 'NONE', ( #21644, #17234 ) ) ;
#17520=CIRCLE ( 'NONE', #1342, 27.14138364107347812 ) ;
#17546=ORIENTED_EDGE ( 'NONE', *, *, #8131, .T. ) ;
#17608=DIRECTION ( 'NONE',  ( 1.000000000000000000, 0.000000000000000000, 0.000000000000000000 ) ) ;
#17628=CARTESIAN_POINT ( 'NONE',  ( -94.10404323627655288, -13.18023274290474767, -19.99999999999997868 ) ) ;
#17640=ORIENTED_EDGE ( 'NONE', *, *, #3591, .F. ) ;
#17723=AXIS2_PLACEMENT_3D ( 'NONE', #12522, #16147, #17901 ) ;
#17747=ORIENTED_EDGE ( 'NONE', *, *, #13847, .T. ) ;
#17793=LINE ( 'NONE', #4350, #20700 ) ;
#17882=EDGE_LOOP ( 'NONE', ( #6194, #18799, #8195, #18742 ) ) ;
#17901=DIRECTION ( 'NONE',  ( -1.000000000000000000, 0.000000000000000000, 0.000000000000000000 ) ) ;
#18026=EDGE_LOOP ( 'NONE', ( #13694, #17747, #19102, #896 ) ) ;
#18047=CARTESIAN_POINT ( 'NONE',  ( -101.1064508287285832, 10.96617311717548660, 4.000000000000021316 ) ) ;
#18079=AXIS2_PLACEMENT_3D ( 'NONE', #6114, #7789, #17474 ) ;
#18118=ADVANCED_FACE ( 'NONE', ( #13280 ), #9866, .F. ) ;
#18173=VECTOR ( 'NONE', #2733, 1000.000000000000114 ) ;
#18203=CARTESIAN_POINT ( 'NONE',  ( -143.7724355939531904, 531.4176628826018032, 4.000000000000021316 ) ) ;
#18227=DIRECTION ( 'NONE',  ( 0.2803088796301150820, -0.9599098561846886035, 0.000000000000000000 ) ) ;
#18346=DIRECTION ( 'NONE',  ( 0.9609502660100632809, 0.2767211344570352782, -0.000000000000000000 ) ) ;
#18358=CARTESIAN_POINT ( 'NONE',  ( -97.23064952102208736, 13.78046159333444720, 4.000000000000021316 ) ) ;
#18383=AXIS2_PLACEMENT_3D ( 'NONE', #11618, #18346, #9978 ) ;
#18388=VECTOR ( 'NONE', #4562, 1000.000000000000000 ) ;
#18710=LINE ( 'NONE', #1954, #7678 ) ;
#18742=ORIENTED_EDGE ( 'NONE', *, *, #4231, .T. ) ;
#18799=ORIENTED_EDGE ( 'NONE', *, *, #9010, .F. ) ;
#18884=ADVANCED_FACE ( 'NONE', ( #21387 ), #14646, .F. ) ;
#18911=DIRECTION ( 'NONE',  ( 0.9609212714474144601, 0.2768218020313508165, 0.000000000000000000 ) ) ;
#18974=DIRECTION ( 'NONE',  ( 1.000000000000000000, 0.000000000000000000, 0.000000000000000000 ) ) ;
#19024=FILL_AREA_STYLE_COLOUR ( '', #20072 ) ;
#19102=ORIENTED_EDGE ( 'NONE', *, *, #14965, .T. ) ;
#19103=DIRECTION ( 'NONE',  ( 1.000000000000000000, 0.000000000000000000, 0.000000000000000000 ) ) ;
#19159=FACE_OUTER_BOUND ( 'NONE', #625, .T. ) ;
#19168=AXIS2_PLACEMENT_3D ( 'NONE', #16190, #11127, #4508 ) ;
#19204=ORIENTED_EDGE ( 'NONE', *, *, #5555, .F. ) ;
#19275=CARTESIAN_POINT ( 'NONE',  ( 151.4773229304660731, 84.89323405393692212, -19.99999999999997868 ) ) ;
#19308=EDGE_LOOP ( 'NONE', ( #9238, #14202, #3942, #4383, #1716, #8833, #9364, #15008 ) ) ;
#19329=CIRCLE ( 'NONE', #10203, 10.00000000000000888 ) ;
#19462=LINE ( 'NONE', #11403, #13301 ) ;
#19546=CARTESIAN_POINT ( 'NONE',  ( -23.27144139456156324, -18.88988604584387332, 4.000000000000021316 ) ) ;
#19571=EDGE_CURVE ( 'NONE', #20969, #9506, #21142, .T. ) ;
#19604=DIRECTION ( 'NONE',  ( -1.000000000000000000, 0.000000000000000000, 0.000000000000000000 ) ) ;
#19647=ADVANCED_FACE ( 'NONE', ( #12649 ), #964, .F. ) ;
#19774=EDGE_CURVE ( 'NONE', #4183, #2361, #17249, .T. ) ;
#19794=ORIENTED_EDGE ( 'NONE', *, *, #6609, .T. ) ;
#19808=CARTESIAN_POINT ( 'NONE',  ( -97.23064952102208736, 13.78046159333444720, -19.99999999999997868 ) ) ;
#19854=CIRCLE ( 'NONE', #18079, 27.14138364107347812 ) ;
#19881=DIRECTION ( 'NONE',  ( -0.9609212714474144601, -0.2768218020313507610, 0.000000000000000000 ) ) ;
#19910=DIRECTION ( 'NONE',  ( -1.000000000000000000, 0.000000000000000000, 0.000000000000000000 ) ) ;
#19998=ORIENTED_EDGE ( 'NONE', *, *, #15163, .F. ) ;
#20009=PLANE ( 'NONE',  #9038 ) ;
#20028=ORIENTED_EDGE ( 'NONE', *, *, #5555, .T. ) ;
#20056=VECTOR ( 'NONE', #20647, 999.9999999999998863 ) ;
#20072=COLOUR_RGB ( '', 0.08235294, 0.09019608, 0.10196078) ;
#20146=DIRECTION ( 'NONE',  ( 0.000000000000000000, 0.000000000000000000, 1.000000000000000000 ) ) ;
#20163=EDGE_CURVE ( 'NONE', #15137, #21430, #13803, .T. ) ;
#20202=DIRECTION ( 'NONE',  ( 0.000000000000000000, 0.000000000000000000, 1.000000000000000000 ) ) ;
#20224=ADVANCED_FACE ( 'NONE', ( #1307 ), #4831, .F. ) ;
#20229=DIRECTION ( 'NONE',  ( 1.000000000000000000, 0.000000000000000000, -0.000000000000000000 ) ) ;
#20301=AXIS2_PLACEMENT_3D ( 'NONE', #20753, #12365, #19103 ) ;
#20358=DIRECTION ( 'NONE',  ( 0.000000000000000000, 0.000000000000000000, 1.000000000000000000 ) ) ;
#20431=ORIENTED_EDGE ( 'NONE', *, *, #11604, .F. ) ;
#20552=DIRECTION ( 'NONE',  ( 0.000000000000000000, 0.000000000000000000, 1.000000000000000000 ) ) ;
#20583=CYLINDRICAL_SURFACE ( 'NONE', #975, 576.1986910693910886 ) ;
#20647=DIRECTION ( 'NONE',  ( 0.2767211344570353337, -0.9609502660100633920, 0.000000000000000000 ) ) ;
#20673=ORIENTED_EDGE ( 'NONE', *, *, #15163, .T. ) ;
#20681=DIRECTION ( 'NONE',  ( 1.000000000000000000, 0.000000000000000000, 0.000000000000000000 ) ) ;
#20700=VECTOR ( 'NONE', #14062, 1000.000000000000114 ) ;
#20753=CARTESIAN_POINT ( 'NONE',  ( -91.10645082872859746, 10.96617311717548660, 4.000000000000021316 ) ) ;
#20891=PLANE ( 'NONE',  #9240 ) ;
#20915=PRODUCT_DEFINITION ( 'UNKNOWN', '', #3886, #10389 ) ;
#20926=( LENGTH_UNIT ( ) NAMED_UNIT ( * ) SI_UNIT ( .MILLI., .METRE. ) );
#20969=VERTEX_POINT ( 'NONE', #8018 ) ;
#20984=VECTOR ( 'NONE', #17228, 1000.000000000000000 ) ;
#21045=CARTESIAN_POINT ( 'NONE',  ( -94.10404323627655288, -13.18023274290474767, -19.99999999999997868 ) ) ;
#21125=ORIENTED_EDGE ( 'NONE', *, *, #13071, .T. ) ;
#21142=LINE ( 'NONE', #6027, #6505 ) ;
#21147=EDGE_CURVE ( 'NONE', #488, #13376, #19329, .T. ) ;
#21173=ORIENTED_EDGE ( 'NONE', *, *, #6919, .T. ) ;
#21226=CARTESIAN_POINT ( 'NONE',  ( -38.21168032741934439, -23.19216891395253910, 4.000000000000021316 ) ) ;
#21267=CARTESIAN_POINT ( 'NONE',  ( -23.27144139456156324, -18.88988604584387332, 4.000000000000021316 ) ) ;
#21270=CARTESIAN_POINT ( 'NONE',  ( -91.10645082872859746, 10.96617311717548660, 4.000000000000021316 ) ) ;
#21297=EDGE_LOOP ( 'NONE', ( #7582, #16362, #337, #2150 ) ) ;
#21350=EDGE_CURVE ( 'NONE', #3570, #951, #16507, .T. ) ;
#21387=FACE_OUTER_BOUND ( 'NONE', #17882, .T. ) ;
#21430=VERTEX_POINT ( 'NONE', #5357 ) ;
#21516=EDGE_LOOP ( 'NONE', ( #570, #9933, #17074, #7501 ) ) ;
#21529=MANIFOLD_SOLID_BREP ( 'Boss-Extrude4', #375 ) ;
#21538=CARTESIAN_POINT ( 'NONE',  ( -91.10645082872859746, 10.96617311717548660, -19.99999999999997868 ) ) ;
#21544=DIRECTION ( 'NONE',  ( 0.2767211344570353337, -0.9609502660100633920, 0.000000000000000000 ) ) ;
#21556=CIRCLE ( 'NONE', #12041, 27.14138364107347812 ) ;
#21577=LINE ( 'NONE', #21798, #5462 ) ;
#21644=ORIENTED_EDGE ( 'NONE', *, *, #1717, .T. ) ;
#21677=DIRECTION ( 'NONE',  ( -0.000000000000000000, -0.000000000000000000, -1.000000000000000000 ) ) ;
#21745=DIRECTION ( 'NONE',  ( -0.000000000000000000, -0.000000000000000000, -1.000000000000000000 ) ) ;
#21798=CARTESIAN_POINT ( 'NONE',  ( -104.7439762501682736, 39.86119447055682485, 4.000000000000021316 ) ) ;
#21813=VERTEX_POINT ( 'NONE', #5385 ) ;
ENDSEC;
END-ISO-10303-21;
